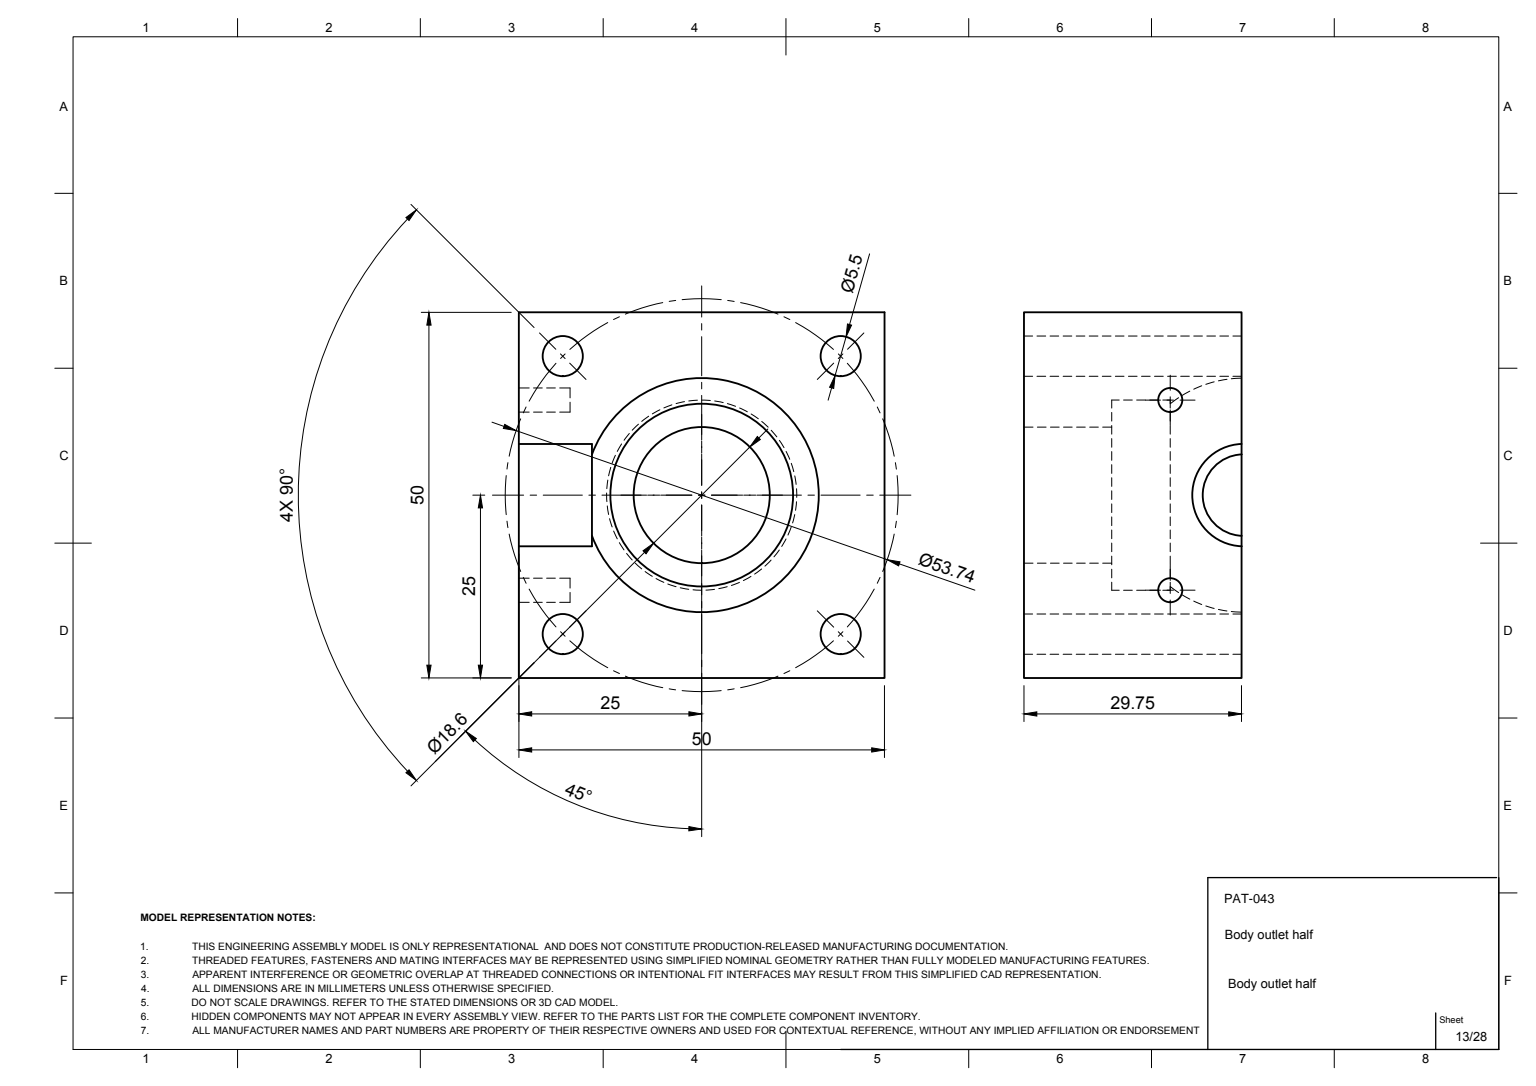
ISO-10303-21;
HEADER;
/* Generated by software containing ST-Developer
 * from STEP Tools, Inc. (www.steptools.com) 
 */

FILE_DESCRIPTION(
/* description */ ('Four-valve pipe header'),
/* implementation_level */ '2;1');

FILE_NAME(
/* name */ 'Body outlet half.step',
/* time_stamp */ '2026-10-29T16:56:19-07:00',
/* author */ (''),
/* organization */ (''),
/* preprocessor_version */ 'ST-DEVELOPER v20.2',
/* originating_system */ 'Autodesk Translation Framework v15.17.0.0',
/* authorisation */ '');

FILE_SCHEMA (('AUTOMOTIVE_DESIGN { 1 0 10303 214 3 1 1 }'));
ENDSEC;

DATA;
#10=MECHANICAL_DESIGN_GEOMETRIC_PRESENTATION_REPRESENTATION('',(#339),#10119);
#243=SPHERICAL_SURFACE('',#6185,1.6);
#287=SHAPE_REPRESENTATION_RELATIONSHIP('SRR','None',#10249,#313);
#313=ADVANCED_BREP_SHAPE_REPRESENTATION('',(#365),#10098);
#339=STYLED_ITEM('',(#10449),#365);
#365=MANIFOLD_SOLID_BREP('Body1',#5585);
#470=FACE_BOUND('',#1258,.T.);
#471=FACE_BOUND('',#1259,.T.);
#472=FACE_BOUND('',#1263,.T.);
#473=FACE_BOUND('',#1265,.T.);
#474=FACE_BOUND('',#1267,.T.);
#475=FACE_BOUND('',#1269,.T.);
#476=FACE_BOUND('',#1270,.T.);
#477=FACE_BOUND('',#1271,.T.);
#478=FACE_BOUND('',#1272,.T.);
#479=FACE_BOUND('',#1273,.T.);
#480=FACE_BOUND('',#1276,.T.);
#481=FACE_BOUND('',#1277,.T.);
#482=FACE_BOUND('',#1278,.T.);
#483=FACE_BOUND('',#1279,.T.);
#608=PLANE('',#6153);
#609=PLANE('',#6157);
#610=PLANE('',#6173);
#611=PLANE('',#6175);
#612=PLANE('',#6182);
#613=PLANE('',#6183);
#614=PLANE('',#6187);
#615=PLANE('',#6188);
#616=PLANE('',#6189);
#617=PLANE('',#6190);
#618=PLANE('',#6191);
#871=FACE_OUTER_BOUND('',#1247,.T.);
#872=FACE_OUTER_BOUND('',#1248,.T.);
#873=FACE_OUTER_BOUND('',#1249,.T.);
#874=FACE_OUTER_BOUND('',#1250,.T.);
#875=FACE_OUTER_BOUND('',#1251,.T.);
#876=FACE_OUTER_BOUND('',#1252,.T.);
#877=FACE_OUTER_BOUND('',#1253,.T.);
#878=FACE_OUTER_BOUND('',#1254,.T.);
#879=FACE_OUTER_BOUND('',#1255,.T.);
#880=FACE_OUTER_BOUND('',#1256,.T.);
#881=FACE_OUTER_BOUND('',#1257,.T.);
#882=FACE_OUTER_BOUND('',#1260,.T.);
#883=FACE_OUTER_BOUND('',#1261,.T.);
#884=FACE_OUTER_BOUND('',#1262,.T.);
#885=FACE_OUTER_BOUND('',#1264,.T.);
#886=FACE_OUTER_BOUND('',#1266,.T.);
#887=FACE_OUTER_BOUND('',#1268,.T.);
#888=FACE_OUTER_BOUND('',#1274,.T.);
#889=FACE_OUTER_BOUND('',#1275,.T.);
#890=FACE_OUTER_BOUND('',#1280,.T.);
#891=FACE_OUTER_BOUND('',#1281,.T.);
#1247=EDGE_LOOP('',(#4307,#4308,#4309,#4310));
#1248=EDGE_LOOP('',(#4311));
#1249=EDGE_LOOP('',(#4312,#4313,#4314,#4315));
#1250=EDGE_LOOP('',(#4316));
#1251=EDGE_LOOP('',(#4317,#4318,#4319,#4320));
#1252=EDGE_LOOP('',(#4321,#4322,#4323,#4324));
#1253=EDGE_LOOP('',(#4325,#4326,#4327,#4328));
#1254=EDGE_LOOP('',(#4329,#4330,#4331,#4332));
#1255=EDGE_LOOP('',(#4333,#4334,#4335,#4336));
#1256=EDGE_LOOP('',(#4337,#4338,#4339,#4340));
#1257=EDGE_LOOP('',(#4341,#4342,#4343,#4344,#4345,#4346));
#1258=EDGE_LOOP('',(#4347));
#1259=EDGE_LOOP('',(#4348));
#1260=EDGE_LOOP('',(#4349,#4350,#4351,#4352));
#1261=EDGE_LOOP('',(#4353,#4354,#4355,#4356));
#1262=EDGE_LOOP('',(#4357));
#1263=EDGE_LOOP('',(#4358));
#1264=EDGE_LOOP('',(#4359));
#1265=EDGE_LOOP('',(#4360));
#1266=EDGE_LOOP('',(#4361,#4362));
#1267=EDGE_LOOP('',(#4363));
#1268=EDGE_LOOP('',(#4364,#4365,#4366,#4367));
#1269=EDGE_LOOP('',(#4368));
#1270=EDGE_LOOP('',(#4369));
#1271=EDGE_LOOP('',(#4370));
#1272=EDGE_LOOP('',(#4371));
#1273=EDGE_LOOP('',(#4372));
#1274=EDGE_LOOP('',(#4373,#4374,#4375,#4376));
#1275=EDGE_LOOP('',(#4377,#4378,#4379,#4380,#4381,#4382,#4383,#4384,#4385,
#4386));
#1276=EDGE_LOOP('',(#4387));
#1277=EDGE_LOOP('',(#4388));
#1278=EDGE_LOOP('',(#4389));
#1279=EDGE_LOOP('',(#4390));
#1280=EDGE_LOOP('',(#4391,#4392,#4393,#4394));
#1281=EDGE_LOOP('',(#4395,#4396,#4397,#4398));
#1664=LINE('',#9059,#2082);
#1665=LINE('',#9066,#2083);
#1666=LINE('',#9073,#2084);
#1667=LINE('',#9079,#2085);
#1668=LINE('',#9085,#2086);
#1669=LINE('',#9091,#2087);
#1670=LINE('',#9096,#2088);
#1671=LINE('',#9100,#2089);
#1672=LINE('',#9104,#2090);
#1673=LINE('',#9107,#2091);
#1674=LINE('',#9110,#2092);
#1675=LINE('',#9112,#2093);
#1676=LINE('',#9114,#2094);
#1677=LINE('',#9116,#2095);
#1678=LINE('',#9117,#2096);
#1679=LINE('',#9122,#2097);
#1680=LINE('',#9128,#2098);
#1681=LINE('',#9139,#2099);
#1682=LINE('',#9140,#2100);
#1683=LINE('',#9141,#2101);
#1684=LINE('',#9144,#2102);
#1685=LINE('',#9145,#2103);
#1686=LINE('',#9148,#2104);
#1687=LINE('',#9149,#2105);
#1688=LINE('',#9151,#2106);
#2082=VECTOR('',#7227,0.165);
#2083=VECTOR('',#7236,0.165);
#2084=VECTOR('',#7245,0.275);
#2085=VECTOR('',#7252,0.275);
#2086=VECTOR('',#7259,0.275);
#2087=VECTOR('',#7266,0.275);
#2088=VECTOR('',#7271,1.);
#2089=VECTOR('',#7274,1.);
#2090=VECTOR('',#7279,1.);
#2091=VECTOR('',#7282,1.);
#2092=VECTOR('',#7285,1.);
#2093=VECTOR('',#7286,1.);
#2094=VECTOR('',#7287,1.);
#2095=VECTOR('',#7288,1.);
#2096=VECTOR('',#7289,1.);
#2097=VECTOR('',#7294,0.93);
#2098=VECTOR('',#7301,1.3);
#2099=VECTOR('',#7316,1.);
#2100=VECTOR('',#7317,1.);
#2101=VECTOR('',#7318,1.);
#2102=VECTOR('',#7321,1.);
#2103=VECTOR('',#7322,1.);
#2104=VECTOR('',#7325,1.);
#2105=VECTOR('',#7326,1.);
#2106=VECTOR('',#7329,1.);
#2445=CIRCLE('',#6151,0.165);
#2446=CIRCLE('',#6152,0.165);
#2447=CIRCLE('',#6155,0.165);
#2448=CIRCLE('',#6156,0.165);
#2449=CIRCLE('',#6159,0.275);
#2450=CIRCLE('',#6160,0.275);
#2451=CIRCLE('',#6162,0.275);
#2452=CIRCLE('',#6163,0.275);
#2453=CIRCLE('',#6165,0.275);
#2454=CIRCLE('',#6166,0.275);
#2455=CIRCLE('',#6168,0.275);
#2456=CIRCLE('',#6169,0.275);
#2457=CIRCLE('',#6171,0.7);
#2458=CIRCLE('',#6172,0.7);
#2459=CIRCLE('',#6174,0.556776436283003);
#2460=CIRCLE('',#6177,0.93);
#2461=CIRCLE('',#6178,0.93);
#2462=CIRCLE('',#6180,1.3);
#2463=CIRCLE('',#6181,1.3);
#2464=CIRCLE('',#6184,1.24899959967968);
#2465=CIRCLE('',#6186,1.59980467557762);
#2763=VERTEX_POINT('',#9056);
#2764=VERTEX_POINT('',#9058);
#2765=VERTEX_POINT('',#9063);
#2766=VERTEX_POINT('',#9065);
#2767=VERTEX_POINT('',#9070);
#2768=VERTEX_POINT('',#9072);
#2769=VERTEX_POINT('',#9076);
#2770=VERTEX_POINT('',#9078);
#2771=VERTEX_POINT('',#9082);
#2772=VERTEX_POINT('',#9084);
#2773=VERTEX_POINT('',#9088);
#2774=VERTEX_POINT('',#9090);
#2775=VERTEX_POINT('',#9094);
#2776=VERTEX_POINT('',#9095);
#2777=VERTEX_POINT('',#9097);
#2778=VERTEX_POINT('',#9099);
#2779=VERTEX_POINT('',#9103);
#2780=VERTEX_POINT('',#9105);
#2781=VERTEX_POINT('',#9109);
#2782=VERTEX_POINT('',#9111);
#2783=VERTEX_POINT('',#9113);
#2784=VERTEX_POINT('',#9115);
#2785=VERTEX_POINT('',#9119);
#2786=VERTEX_POINT('',#9121);
#2787=VERTEX_POINT('',#9125);
#2788=VERTEX_POINT('',#9127);
#2789=VERTEX_POINT('',#9132);
#2790=VERTEX_POINT('',#9137);
#2791=VERTEX_POINT('',#9138);
#2792=VERTEX_POINT('',#9143);
#2793=VERTEX_POINT('',#9147);
#3320=EDGE_CURVE('',#2763,#2763,#2445,.T.);
#3321=EDGE_CURVE('',#2763,#2764,#1664,.T.);
#3322=EDGE_CURVE('',#2764,#2764,#2446,.T.);
#3323=EDGE_CURVE('',#2765,#2765,#2447,.T.);
#3324=EDGE_CURVE('',#2765,#2766,#1665,.T.);
#3325=EDGE_CURVE('',#2766,#2766,#2448,.T.);
#3326=EDGE_CURVE('',#2767,#2767,#2449,.T.);
#3327=EDGE_CURVE('',#2767,#2768,#1666,.T.);
#3328=EDGE_CURVE('',#2768,#2768,#2450,.T.);
#3329=EDGE_CURVE('',#2769,#2769,#2451,.T.);
#3330=EDGE_CURVE('',#2769,#2770,#1667,.T.);
#3331=EDGE_CURVE('',#2770,#2770,#2452,.T.);
#3332=EDGE_CURVE('',#2771,#2771,#2453,.T.);
#3333=EDGE_CURVE('',#2771,#2772,#1668,.T.);
#3334=EDGE_CURVE('',#2772,#2772,#2454,.T.);
#3335=EDGE_CURVE('',#2773,#2773,#2455,.T.);
#3336=EDGE_CURVE('',#2773,#2774,#1669,.T.);
#3337=EDGE_CURVE('',#2774,#2774,#2456,.T.);
#3338=EDGE_CURVE('',#2775,#2776,#1670,.T.);
#3339=EDGE_CURVE('',#2777,#2775,#2457,.T.);
#3340=EDGE_CURVE('',#2778,#2777,#1671,.T.);
#3341=EDGE_CURVE('',#2776,#2778,#2458,.T.);
#3342=EDGE_CURVE('',#2779,#2775,#1672,.T.);
#3343=EDGE_CURVE('',#2780,#2779,#2459,.T.);
#3344=EDGE_CURVE('',#2777,#2780,#1673,.T.);
#3345=EDGE_CURVE('',#2778,#2781,#1674,.T.);
#3346=EDGE_CURVE('',#2781,#2782,#1675,.T.);
#3347=EDGE_CURVE('',#2782,#2783,#1676,.T.);
#3348=EDGE_CURVE('',#2783,#2784,#1677,.T.);
#3349=EDGE_CURVE('',#2784,#2776,#1678,.T.);
#3350=EDGE_CURVE('',#2785,#2785,#2460,.T.);
#3351=EDGE_CURVE('',#2785,#2786,#1679,.T.);
#3352=EDGE_CURVE('',#2786,#2786,#2461,.T.);
#3353=EDGE_CURVE('',#2787,#2787,#2462,.T.);
#3354=EDGE_CURVE('',#2787,#2788,#1680,.T.);
#3355=EDGE_CURVE('',#2788,#2788,#2463,.T.);
#3356=EDGE_CURVE('',#2789,#2789,#2464,.T.);
#3357=EDGE_CURVE('',#2780,#2779,#2465,.T.);
#3358=EDGE_CURVE('',#2790,#2791,#1681,.T.);
#3359=EDGE_CURVE('',#2791,#2783,#1682,.T.);
#3360=EDGE_CURVE('',#2790,#2782,#1683,.T.);
#3361=EDGE_CURVE('',#2792,#2790,#1684,.T.);
#3362=EDGE_CURVE('',#2792,#2781,#1685,.T.);
#3363=EDGE_CURVE('',#2793,#2784,#1686,.T.);
#3364=EDGE_CURVE('',#2793,#2792,#1687,.T.);
#3365=EDGE_CURVE('',#2791,#2793,#1688,.T.);
#4307=ORIENTED_EDGE('',*,*,#3320,.F.);
#4308=ORIENTED_EDGE('',*,*,#3321,.T.);
#4309=ORIENTED_EDGE('',*,*,#3322,.F.);
#4310=ORIENTED_EDGE('',*,*,#3321,.F.);
#4311=ORIENTED_EDGE('',*,*,#3320,.T.);
#4312=ORIENTED_EDGE('',*,*,#3323,.F.);
#4313=ORIENTED_EDGE('',*,*,#3324,.T.);
#4314=ORIENTED_EDGE('',*,*,#3325,.F.);
#4315=ORIENTED_EDGE('',*,*,#3324,.F.);
#4316=ORIENTED_EDGE('',*,*,#3323,.T.);
#4317=ORIENTED_EDGE('',*,*,#3326,.F.);
#4318=ORIENTED_EDGE('',*,*,#3327,.T.);
#4319=ORIENTED_EDGE('',*,*,#3328,.F.);
#4320=ORIENTED_EDGE('',*,*,#3327,.F.);
#4321=ORIENTED_EDGE('',*,*,#3329,.F.);
#4322=ORIENTED_EDGE('',*,*,#3330,.T.);
#4323=ORIENTED_EDGE('',*,*,#3331,.F.);
#4324=ORIENTED_EDGE('',*,*,#3330,.F.);
#4325=ORIENTED_EDGE('',*,*,#3332,.F.);
#4326=ORIENTED_EDGE('',*,*,#3333,.T.);
#4327=ORIENTED_EDGE('',*,*,#3334,.F.);
#4328=ORIENTED_EDGE('',*,*,#3333,.F.);
#4329=ORIENTED_EDGE('',*,*,#3335,.F.);
#4330=ORIENTED_EDGE('',*,*,#3336,.T.);
#4331=ORIENTED_EDGE('',*,*,#3337,.F.);
#4332=ORIENTED_EDGE('',*,*,#3336,.F.);
#4333=ORIENTED_EDGE('',*,*,#3338,.F.);
#4334=ORIENTED_EDGE('',*,*,#3339,.F.);
#4335=ORIENTED_EDGE('',*,*,#3340,.F.);
#4336=ORIENTED_EDGE('',*,*,#3341,.F.);
#4337=ORIENTED_EDGE('',*,*,#3342,.F.);
#4338=ORIENTED_EDGE('',*,*,#3343,.F.);
#4339=ORIENTED_EDGE('',*,*,#3344,.F.);
#4340=ORIENTED_EDGE('',*,*,#3339,.T.);
#4341=ORIENTED_EDGE('',*,*,#3341,.T.);
#4342=ORIENTED_EDGE('',*,*,#3345,.T.);
#4343=ORIENTED_EDGE('',*,*,#3346,.T.);
#4344=ORIENTED_EDGE('',*,*,#3347,.T.);
#4345=ORIENTED_EDGE('',*,*,#3348,.T.);
#4346=ORIENTED_EDGE('',*,*,#3349,.T.);
#4347=ORIENTED_EDGE('',*,*,#3322,.T.);
#4348=ORIENTED_EDGE('',*,*,#3325,.T.);
#4349=ORIENTED_EDGE('',*,*,#3350,.F.);
#4350=ORIENTED_EDGE('',*,*,#3351,.T.);
#4351=ORIENTED_EDGE('',*,*,#3352,.F.);
#4352=ORIENTED_EDGE('',*,*,#3351,.F.);
#4353=ORIENTED_EDGE('',*,*,#3353,.F.);
#4354=ORIENTED_EDGE('',*,*,#3354,.T.);
#4355=ORIENTED_EDGE('',*,*,#3355,.T.);
#4356=ORIENTED_EDGE('',*,*,#3354,.F.);
#4357=ORIENTED_EDGE('',*,*,#3355,.F.);
#4358=ORIENTED_EDGE('',*,*,#3350,.T.);
#4359=ORIENTED_EDGE('',*,*,#3353,.T.);
#4360=ORIENTED_EDGE('',*,*,#3356,.F.);
#4361=ORIENTED_EDGE('',*,*,#3343,.T.);
#4362=ORIENTED_EDGE('',*,*,#3357,.F.);
#4363=ORIENTED_EDGE('',*,*,#3356,.T.);
#4364=ORIENTED_EDGE('',*,*,#3358,.T.);
#4365=ORIENTED_EDGE('',*,*,#3359,.T.);
#4366=ORIENTED_EDGE('',*,*,#3347,.F.);
#4367=ORIENTED_EDGE('',*,*,#3360,.F.);
#4368=ORIENTED_EDGE('',*,*,#3352,.T.);
#4369=ORIENTED_EDGE('',*,*,#3337,.T.);
#4370=ORIENTED_EDGE('',*,*,#3334,.T.);
#4371=ORIENTED_EDGE('',*,*,#3331,.T.);
#4372=ORIENTED_EDGE('',*,*,#3328,.T.);
#4373=ORIENTED_EDGE('',*,*,#3361,.T.);
#4374=ORIENTED_EDGE('',*,*,#3360,.T.);
#4375=ORIENTED_EDGE('',*,*,#3346,.F.);
#4376=ORIENTED_EDGE('',*,*,#3362,.F.);
#4377=ORIENTED_EDGE('',*,*,#3338,.T.);
#4378=ORIENTED_EDGE('',*,*,#3349,.F.);
#4379=ORIENTED_EDGE('',*,*,#3363,.F.);
#4380=ORIENTED_EDGE('',*,*,#3364,.T.);
#4381=ORIENTED_EDGE('',*,*,#3362,.T.);
#4382=ORIENTED_EDGE('',*,*,#3345,.F.);
#4383=ORIENTED_EDGE('',*,*,#3340,.T.);
#4384=ORIENTED_EDGE('',*,*,#3344,.T.);
#4385=ORIENTED_EDGE('',*,*,#3357,.T.);
#4386=ORIENTED_EDGE('',*,*,#3342,.T.);
#4387=ORIENTED_EDGE('',*,*,#3326,.T.);
#4388=ORIENTED_EDGE('',*,*,#3329,.T.);
#4389=ORIENTED_EDGE('',*,*,#3332,.T.);
#4390=ORIENTED_EDGE('',*,*,#3335,.T.);
#4391=ORIENTED_EDGE('',*,*,#3365,.T.);
#4392=ORIENTED_EDGE('',*,*,#3363,.T.);
#4393=ORIENTED_EDGE('',*,*,#3348,.F.);
#4394=ORIENTED_EDGE('',*,*,#3359,.F.);
#4395=ORIENTED_EDGE('',*,*,#3365,.F.);
#4396=ORIENTED_EDGE('',*,*,#3358,.F.);
#4397=ORIENTED_EDGE('',*,*,#3361,.F.);
#4398=ORIENTED_EDGE('',*,*,#3364,.F.);
#5197=CYLINDRICAL_SURFACE('',#6150,0.165);
#5198=CYLINDRICAL_SURFACE('',#6154,0.165);
#5199=CYLINDRICAL_SURFACE('',#6158,0.275);
#5200=CYLINDRICAL_SURFACE('',#6161,0.275);
#5201=CYLINDRICAL_SURFACE('',#6164,0.275);
#5202=CYLINDRICAL_SURFACE('',#6167,0.275);
#5203=CYLINDRICAL_SURFACE('',#6170,0.7);
#5204=CYLINDRICAL_SURFACE('',#6176,0.93);
#5205=CYLINDRICAL_SURFACE('',#6179,1.3);
#5371=ADVANCED_FACE('',(#871),#5197,.F.);
#5372=ADVANCED_FACE('',(#872),#608,.T.);
#5373=ADVANCED_FACE('',(#873),#5198,.F.);
#5374=ADVANCED_FACE('',(#874),#609,.T.);
#5375=ADVANCED_FACE('',(#875),#5199,.F.);
#5376=ADVANCED_FACE('',(#876),#5200,.F.);
#5377=ADVANCED_FACE('',(#877),#5201,.F.);
#5378=ADVANCED_FACE('',(#878),#5202,.F.);
#5379=ADVANCED_FACE('',(#879),#5203,.F.);
#5380=ADVANCED_FACE('',(#880),#610,.T.);
#5381=ADVANCED_FACE('',(#881,#470,#471),#611,.T.);
#5382=ADVANCED_FACE('',(#882),#5204,.F.);
#5383=ADVANCED_FACE('',(#883),#5205,.F.);
#5384=ADVANCED_FACE('',(#884,#472),#612,.F.);
#5385=ADVANCED_FACE('',(#885,#473),#613,.T.);
#5386=ADVANCED_FACE('',(#886,#474),#243,.F.);
#5387=ADVANCED_FACE('',(#887,#475,#476,#477,#478,#479),#614,.T.);
#5388=ADVANCED_FACE('',(#888),#615,.T.);
#5389=ADVANCED_FACE('',(#889,#480,#481,#482,#483),#616,.T.);
#5390=ADVANCED_FACE('',(#890),#617,.T.);
#5391=ADVANCED_FACE('',(#891),#618,.F.);
#5585=CLOSED_SHELL('',(#5371,#5372,#5373,#5374,#5375,#5376,#5377,#5378,
#5379,#5380,#5381,#5382,#5383,#5384,#5385,#5386,#5387,#5388,#5389,#5390,
#5391));
#6149=AXIS2_PLACEMENT_3D('',#9054,#7221,#7222);
#6150=AXIS2_PLACEMENT_3D('',#9055,#7223,#7224);
#6151=AXIS2_PLACEMENT_3D('',#9057,#7225,#7226);
#6152=AXIS2_PLACEMENT_3D('',#9060,#7228,#7229);
#6153=AXIS2_PLACEMENT_3D('',#9061,#7230,#7231);
#6154=AXIS2_PLACEMENT_3D('',#9062,#7232,#7233);
#6155=AXIS2_PLACEMENT_3D('',#9064,#7234,#7235);
#6156=AXIS2_PLACEMENT_3D('',#9067,#7237,#7238);
#6157=AXIS2_PLACEMENT_3D('',#9068,#7239,#7240);
#6158=AXIS2_PLACEMENT_3D('',#9069,#7241,#7242);
#6159=AXIS2_PLACEMENT_3D('',#9071,#7243,#7244);
#6160=AXIS2_PLACEMENT_3D('',#9074,#7246,#7247);
#6161=AXIS2_PLACEMENT_3D('',#9075,#7248,#7249);
#6162=AXIS2_PLACEMENT_3D('',#9077,#7250,#7251);
#6163=AXIS2_PLACEMENT_3D('',#9080,#7253,#7254);
#6164=AXIS2_PLACEMENT_3D('',#9081,#7255,#7256);
#6165=AXIS2_PLACEMENT_3D('',#9083,#7257,#7258);
#6166=AXIS2_PLACEMENT_3D('',#9086,#7260,#7261);
#6167=AXIS2_PLACEMENT_3D('',#9087,#7262,#7263);
#6168=AXIS2_PLACEMENT_3D('',#9089,#7264,#7265);
#6169=AXIS2_PLACEMENT_3D('',#9092,#7267,#7268);
#6170=AXIS2_PLACEMENT_3D('',#9093,#7269,#7270);
#6171=AXIS2_PLACEMENT_3D('',#9098,#7272,#7273);
#6172=AXIS2_PLACEMENT_3D('',#9101,#7275,#7276);
#6173=AXIS2_PLACEMENT_3D('',#9102,#7277,#7278);
#6174=AXIS2_PLACEMENT_3D('',#9106,#7280,#7281);
#6175=AXIS2_PLACEMENT_3D('',#9108,#7283,#7284);
#6176=AXIS2_PLACEMENT_3D('',#9118,#7290,#7291);
#6177=AXIS2_PLACEMENT_3D('',#9120,#7292,#7293);
#6178=AXIS2_PLACEMENT_3D('',#9123,#7295,#7296);
#6179=AXIS2_PLACEMENT_3D('',#9124,#7297,#7298);
#6180=AXIS2_PLACEMENT_3D('',#9126,#7299,#7300);
#6181=AXIS2_PLACEMENT_3D('',#9129,#7302,#7303);
#6182=AXIS2_PLACEMENT_3D('',#9130,#7304,#7305);
#6183=AXIS2_PLACEMENT_3D('',#9131,#7306,#7307);
#6184=AXIS2_PLACEMENT_3D('',#9133,#7308,#7309);
#6185=AXIS2_PLACEMENT_3D('',#9134,#7310,#7311);
#6186=AXIS2_PLACEMENT_3D('',#9135,#7312,#7313);
#6187=AXIS2_PLACEMENT_3D('',#9136,#7314,#7315);
#6188=AXIS2_PLACEMENT_3D('',#9142,#7319,#7320);
#6189=AXIS2_PLACEMENT_3D('',#9146,#7323,#7324);
#6190=AXIS2_PLACEMENT_3D('',#9150,#7327,#7328);
#6191=AXIS2_PLACEMENT_3D('',#9152,#7330,#7331);
#7221=DIRECTION('axis',(0.,0.,1.));
#7222=DIRECTION('refdir',(1.,0.,0.));
#7223=DIRECTION('center_axis',(0.,0.,1.));
#7224=DIRECTION('ref_axis',(1.,0.,0.));
#7225=DIRECTION('center_axis',(0.,0.,1.));
#7226=DIRECTION('ref_axis',(1.,0.,0.));
#7227=DIRECTION('',(0.,0.,1.));
#7228=DIRECTION('center_axis',(0.,0.,-1.));
#7229=DIRECTION('ref_axis',(1.,0.,0.));
#7230=DIRECTION('center_axis',(0.,0.,1.));
#7231=DIRECTION('ref_axis',(1.,0.,0.));
#7232=DIRECTION('center_axis',(0.,0.,1.));
#7233=DIRECTION('ref_axis',(1.,0.,0.));
#7234=DIRECTION('center_axis',(0.,0.,1.));
#7235=DIRECTION('ref_axis',(1.,0.,0.));
#7236=DIRECTION('',(0.,0.,1.));
#7237=DIRECTION('center_axis',(0.,0.,-1.));
#7238=DIRECTION('ref_axis',(1.,0.,0.));
#7239=DIRECTION('center_axis',(0.,0.,1.));
#7240=DIRECTION('ref_axis',(1.,0.,0.));
#7241=DIRECTION('center_axis',(0.,1.,0.));
#7242=DIRECTION('ref_axis',(1.,0.,0.));
#7243=DIRECTION('center_axis',(0.,1.,0.));
#7244=DIRECTION('ref_axis',(1.,0.,0.));
#7245=DIRECTION('',(0.,1.,0.));
#7246=DIRECTION('center_axis',(0.,-1.,0.));
#7247=DIRECTION('ref_axis',(1.,0.,0.));
#7248=DIRECTION('center_axis',(0.,1.,0.));
#7249=DIRECTION('ref_axis',(1.,0.,0.));
#7250=DIRECTION('center_axis',(0.,1.,0.));
#7251=DIRECTION('ref_axis',(1.,0.,0.));
#7252=DIRECTION('',(0.,1.,0.));
#7253=DIRECTION('center_axis',(0.,-1.,0.));
#7254=DIRECTION('ref_axis',(1.,0.,0.));
#7255=DIRECTION('center_axis',(0.,1.,0.));
#7256=DIRECTION('ref_axis',(1.,0.,0.));
#7257=DIRECTION('center_axis',(0.,1.,0.));
#7258=DIRECTION('ref_axis',(1.,0.,0.));
#7259=DIRECTION('',(0.,1.,0.));
#7260=DIRECTION('center_axis',(0.,-1.,0.));
#7261=DIRECTION('ref_axis',(1.,0.,0.));
#7262=DIRECTION('center_axis',(0.,1.,0.));
#7263=DIRECTION('ref_axis',(1.,0.,0.));
#7264=DIRECTION('center_axis',(0.,1.,0.));
#7265=DIRECTION('ref_axis',(1.,0.,0.));
#7266=DIRECTION('',(0.,1.,0.));
#7267=DIRECTION('center_axis',(0.,-1.,0.));
#7268=DIRECTION('ref_axis',(1.,0.,0.));
#7269=DIRECTION('center_axis',(0.,0.,1.));
#7270=DIRECTION('ref_axis',(1.,0.,0.));
#7271=DIRECTION('',(0.,0.,1.));
#7272=DIRECTION('center_axis',(0.,0.,1.));
#7273=DIRECTION('ref_axis',(1.,0.,0.));
#7274=DIRECTION('',(0.,0.,-1.));
#7275=DIRECTION('center_axis',(0.,0.,-1.));
#7276=DIRECTION('ref_axis',(1.,0.,0.));
#7277=DIRECTION('center_axis',(0.,0.,1.));
#7278=DIRECTION('ref_axis',(1.,0.,0.));
#7279=DIRECTION('',(-1.,0.,0.));
#7280=DIRECTION('center_axis',(0.,0.,1.));
#7281=DIRECTION('ref_axis',(0.,-1.,0.));
#7282=DIRECTION('',(-1.,0.,0.));
#7283=DIRECTION('center_axis',(0.,0.,1.));
#7284=DIRECTION('ref_axis',(1.,0.,0.));
#7285=DIRECTION('',(1.,0.,0.));
#7286=DIRECTION('',(0.,1.,0.));
#7287=DIRECTION('',(-1.,0.,0.));
#7288=DIRECTION('',(0.,-1.,0.));
#7289=DIRECTION('',(1.,0.,0.));
#7290=DIRECTION('center_axis',(0.,1.,0.));
#7291=DIRECTION('ref_axis',(1.,0.,0.));
#7292=DIRECTION('center_axis',(0.,1.,0.));
#7293=DIRECTION('ref_axis',(1.,0.,0.));
#7294=DIRECTION('',(0.,1.,0.));
#7295=DIRECTION('center_axis',(0.,-1.,0.));
#7296=DIRECTION('ref_axis',(1.,0.,0.));
#7297=DIRECTION('center_axis',(0.,1.,0.));
#7298=DIRECTION('ref_axis',(1.,0.,0.));
#7299=DIRECTION('center_axis',(0.,1.,0.));
#7300=DIRECTION('ref_axis',(1.,0.,0.));
#7301=DIRECTION('',(0.,1.,0.));
#7302=DIRECTION('center_axis',(0.,1.,0.));
#7303=DIRECTION('ref_axis',(1.,0.,0.));
#7304=DIRECTION('center_axis',(0.,1.,0.));
#7305=DIRECTION('ref_axis',(1.,0.,0.));
#7306=DIRECTION('center_axis',(0.,1.,0.));
#7307=DIRECTION('ref_axis',(1.,0.,0.));
#7308=DIRECTION('center_axis',(0.,1.,0.));
#7309=DIRECTION('ref_axis',(0.,0.,1.));
#7310=DIRECTION('center_axis',(6.12323399573677E-17,0.,1.));
#7311=DIRECTION('ref_axis',(1.,0.,0.));
#7312=DIRECTION('center_axis',(0.,1.,0.));
#7313=DIRECTION('ref_axis',(0.,0.,1.));
#7314=DIRECTION('center_axis',(0.,1.,0.));
#7315=DIRECTION('ref_axis',(-1.,0.,0.));
#7316=DIRECTION('',(-1.,0.,0.));
#7317=DIRECTION('',(0.,0.,1.));
#7318=DIRECTION('',(0.,0.,1.));
#7319=DIRECTION('center_axis',(1.,0.,0.));
#7320=DIRECTION('ref_axis',(0.,1.,0.));
#7321=DIRECTION('',(0.,1.,0.));
#7322=DIRECTION('',(0.,0.,1.));
#7323=DIRECTION('center_axis',(0.,-1.,0.));
#7324=DIRECTION('ref_axis',(1.,0.,0.));
#7325=DIRECTION('',(0.,0.,1.));
#7326=DIRECTION('',(1.,0.,0.));
#7327=DIRECTION('center_axis',(-1.,0.,0.));
#7328=DIRECTION('ref_axis',(0.,-1.,0.));
#7329=DIRECTION('',(0.,-1.,0.));
#7330=DIRECTION('center_axis',(0.,0.,1.));
#7331=DIRECTION('ref_axis',(1.,0.,0.));
#9054=CARTESIAN_POINT('',(0.,0.,0.));
#9055=CARTESIAN_POINT('Origin',(-1.3,1.,6.8));
#9056=CARTESIAN_POINT('',(-1.465,1.,6.8));
#9057=CARTESIAN_POINT('Origin',(-1.3,1.,6.8));
#9058=CARTESIAN_POINT('',(-1.465,1.,7.5));
#9059=CARTESIAN_POINT('',(-1.465,1.,6.8));
#9060=CARTESIAN_POINT('Origin',(-1.3,1.,7.5));
#9061=CARTESIAN_POINT('Origin',(-1.3,1.,6.8));
#9062=CARTESIAN_POINT('Origin',(1.3,1.,6.8));
#9063=CARTESIAN_POINT('',(1.135,1.,6.8));
#9064=CARTESIAN_POINT('Origin',(1.3,1.,6.8));
#9065=CARTESIAN_POINT('',(1.135,1.,7.5));
#9066=CARTESIAN_POINT('',(1.135,1.,6.8));
#9067=CARTESIAN_POINT('Origin',(1.3,1.,7.5));
#9068=CARTESIAN_POINT('Origin',(1.3,1.,6.8));
#9069=CARTESIAN_POINT('Origin',(1.9,-3.1,3.1));
#9070=CARTESIAN_POINT('',(1.625,0.0249999999999999,3.1));
#9071=CARTESIAN_POINT('Origin',(1.9,0.0249999999999999,3.1));
#9072=CARTESIAN_POINT('',(1.625,3.,3.1));
#9073=CARTESIAN_POINT('',(1.625,-3.1,3.1));
#9074=CARTESIAN_POINT('Origin',(1.9,3.,3.1));
#9075=CARTESIAN_POINT('Origin',(-1.9,-3.1,6.9));
#9076=CARTESIAN_POINT('',(-2.175,0.0249999999999999,6.9));
#9077=CARTESIAN_POINT('Origin',(-1.9,0.0249999999999999,6.9));
#9078=CARTESIAN_POINT('',(-2.175,3.,6.9));
#9079=CARTESIAN_POINT('',(-2.175,-3.1,6.9));
#9080=CARTESIAN_POINT('Origin',(-1.9,3.,6.9));
#9081=CARTESIAN_POINT('Origin',(-1.9,-3.1,3.1));
#9082=CARTESIAN_POINT('',(-2.175,0.0249999999999999,3.1));
#9083=CARTESIAN_POINT('Origin',(-1.9,0.0249999999999999,3.1));
#9084=CARTESIAN_POINT('',(-2.175,3.,3.1));
#9085=CARTESIAN_POINT('',(-2.175,-3.1,3.1));
#9086=CARTESIAN_POINT('Origin',(-1.9,3.,3.1));
#9087=CARTESIAN_POINT('Origin',(1.9,-3.1,6.9));
#9088=CARTESIAN_POINT('',(1.625,0.0249999999999999,6.9));
#9089=CARTESIAN_POINT('Origin',(1.9,0.0249999999999999,6.9));
#9090=CARTESIAN_POINT('',(1.625,3.,6.9));
#9091=CARTESIAN_POINT('',(1.625,-3.1,6.9));
#9092=CARTESIAN_POINT('Origin',(1.9,3.,6.9));
#9093=CARTESIAN_POINT('Origin',(0.,0.,6.5));
#9094=CARTESIAN_POINT('',(-0.699553428981661,0.025,6.5));
#9095=CARTESIAN_POINT('',(-0.699553428981661,0.025,7.5));
#9096=CARTESIAN_POINT('',(-0.699553428981661,0.025,6.5));
#9097=CARTESIAN_POINT('',(0.699553428981661,0.025,6.5));
#9098=CARTESIAN_POINT('Origin',(0.,0.,6.5));
#9099=CARTESIAN_POINT('',(0.699553428981661,0.025,7.5));
#9100=CARTESIAN_POINT('',(0.699553428981661,0.025,6.5));
#9101=CARTESIAN_POINT('Origin',(0.,0.,7.5));
#9102=CARTESIAN_POINT('Origin',(0.,0.,6.5));
#9103=CARTESIAN_POINT('',(-0.556214886532175,0.025,6.5));
#9104=CARTESIAN_POINT('',(-1.25,0.025,6.5));
#9105=CARTESIAN_POINT('',(0.556214886532175,0.025,6.5));
#9106=CARTESIAN_POINT('Origin',(0.,0.,6.5));
#9107=CARTESIAN_POINT('',(-1.25,0.025,6.5));
#9108=CARTESIAN_POINT('Origin',(0.,1.5125,7.5));
#9109=CARTESIAN_POINT('',(2.5,0.0249999999999999,7.5));
#9110=CARTESIAN_POINT('',(-2.5,0.025,7.5));
#9111=CARTESIAN_POINT('',(2.5,3.,7.5));
#9112=CARTESIAN_POINT('',(2.5,0.025,7.5));
#9113=CARTESIAN_POINT('',(-2.5,3.,7.5));
#9114=CARTESIAN_POINT('',(2.5,3.,7.5));
#9115=CARTESIAN_POINT('',(-2.5,0.0249999999999999,7.5));
#9116=CARTESIAN_POINT('',(-2.5,3.,7.5));
#9117=CARTESIAN_POINT('',(-2.5,0.025,7.5));
#9118=CARTESIAN_POINT('Origin',(0.,1.8,5.));
#9119=CARTESIAN_POINT('',(-0.93,1.8,5.));
#9120=CARTESIAN_POINT('Origin',(0.,1.8,5.));
#9121=CARTESIAN_POINT('',(-0.93,3.,5.));
#9122=CARTESIAN_POINT('',(-0.93,1.8,5.));
#9123=CARTESIAN_POINT('Origin',(0.,3.,5.));
#9124=CARTESIAN_POINT('Origin',(0.,1.,5.));
#9125=CARTESIAN_POINT('',(-1.3,1.,5.));
#9126=CARTESIAN_POINT('Origin',(0.,1.,5.));
#9127=CARTESIAN_POINT('',(-1.3,1.8,5.));
#9128=CARTESIAN_POINT('',(-1.3,1.,5.));
#9129=CARTESIAN_POINT('Origin',(0.,1.8,5.));
#9130=CARTESIAN_POINT('Origin',(0.,1.8,5.));
#9131=CARTESIAN_POINT('Origin',(0.,1.,5.));
#9132=CARTESIAN_POINT('',(-1.52958336188405E-16,1.,3.75100040032032));
#9133=CARTESIAN_POINT('Origin',(0.,1.,5.));
#9134=CARTESIAN_POINT('Origin',(0.,0.,5.));
#9135=CARTESIAN_POINT('Origin',(0.,0.025,5.));
#9136=CARTESIAN_POINT('Origin',(2.5,3.,2.5));
#9137=CARTESIAN_POINT('',(2.5,3.,2.5));
#9138=CARTESIAN_POINT('',(-2.5,3.,2.5));
#9139=CARTESIAN_POINT('',(2.5,3.,2.5));
#9140=CARTESIAN_POINT('',(-2.5,3.,2.5));
#9141=CARTESIAN_POINT('',(2.5,3.,2.5));
#9142=CARTESIAN_POINT('Origin',(2.5,0.025,2.5));
#9143=CARTESIAN_POINT('',(2.5,0.025,2.5));
#9144=CARTESIAN_POINT('',(2.5,0.025,2.5));
#9145=CARTESIAN_POINT('',(2.5,0.025,2.5));
#9146=CARTESIAN_POINT('Origin',(-2.5,0.025,2.5));
#9147=CARTESIAN_POINT('',(-2.5,0.0249999999999999,2.5));
#9148=CARTESIAN_POINT('',(-2.5,0.0249999999999999,2.5));
#9149=CARTESIAN_POINT('',(-2.5,0.025,2.5));
#9150=CARTESIAN_POINT('Origin',(-2.5,3.,2.5));
#9151=CARTESIAN_POINT('',(-2.5,3.,2.5));
#9152=CARTESIAN_POINT('Origin',(0.,1.5125,2.5));
#10067=UNCERTAINTY_MEASURE_WITH_UNIT(LENGTH_MEASURE(0.001),#10120,
'DISTANCE_ACCURACY_VALUE',
'Maximum model space distance between geometric entities at asserted c
onnectivities');
#10088=UNCERTAINTY_MEASURE_WITH_UNIT(LENGTH_MEASURE(0.001),#10120,
'DISTANCE_ACCURACY_VALUE',
'Maximum model space distance between geometric entities at asserted c
onnectivities');
#10098=(
GEOMETRIC_REPRESENTATION_CONTEXT(3)
GLOBAL_UNCERTAINTY_ASSIGNED_CONTEXT((#10067))
GLOBAL_UNIT_ASSIGNED_CONTEXT((#10120,#10122,#10123))
REPRESENTATION_CONTEXT('','3D')
);
#10119=(
GEOMETRIC_REPRESENTATION_CONTEXT(3)
GLOBAL_UNCERTAINTY_ASSIGNED_CONTEXT((#10088))
GLOBAL_UNIT_ASSIGNED_CONTEXT((#10120,#10122,#10123))
REPRESENTATION_CONTEXT('','3D')
);
#10120=(
LENGTH_UNIT()
NAMED_UNIT(*)
SI_UNIT(.CENTI.,.METRE.)
);
#10122=(
NAMED_UNIT(*)
PLANE_ANGLE_UNIT()
SI_UNIT($,.RADIAN.)
);
#10123=(
NAMED_UNIT(*)
SI_UNIT($,.STERADIAN.)
SOLID_ANGLE_UNIT()
);
#10133=SHAPE_DEFINITION_REPRESENTATION(#10163,#10249);
#10163=PRODUCT_DEFINITION_SHAPE('',$,#10280);
#10249=SHAPE_REPRESENTATION('',(#6149),#10098);
#10270=PRODUCT_DEFINITION_CONTEXT('part definition',#10362,'design');
#10280=PRODUCT_DEFINITION('Body outlet half','Body outlet half',#10310,
#10270);
#10310=PRODUCT_DEFINITION_FORMATION('',$,#10373);
#10362=APPLICATION_CONTEXT(
'Core Data for Automotive Mechanical Design Process');
#10363=PRODUCT_CONTEXT('part definition',#10362,'mechanical');
#10373=PRODUCT('Body outlet half','Body outlet half','Body outlet half',
(#10363));
#10443=COLOUR_RGB('Dark Blue',0.08,0.2,0.34);
#10444=FILL_AREA_STYLE_COLOUR('',#10443);
#10445=FILL_AREA_STYLE('',(#10444));
#10446=SURFACE_STYLE_FILL_AREA(#10445);
#10447=SURFACE_SIDE_STYLE('',(#10446));
#10448=SURFACE_STYLE_USAGE(.BOTH.,#10447);
#10449=PRESENTATION_STYLE_ASSIGNMENT((#10448));
ENDSEC;
END-ISO-10303-21;
